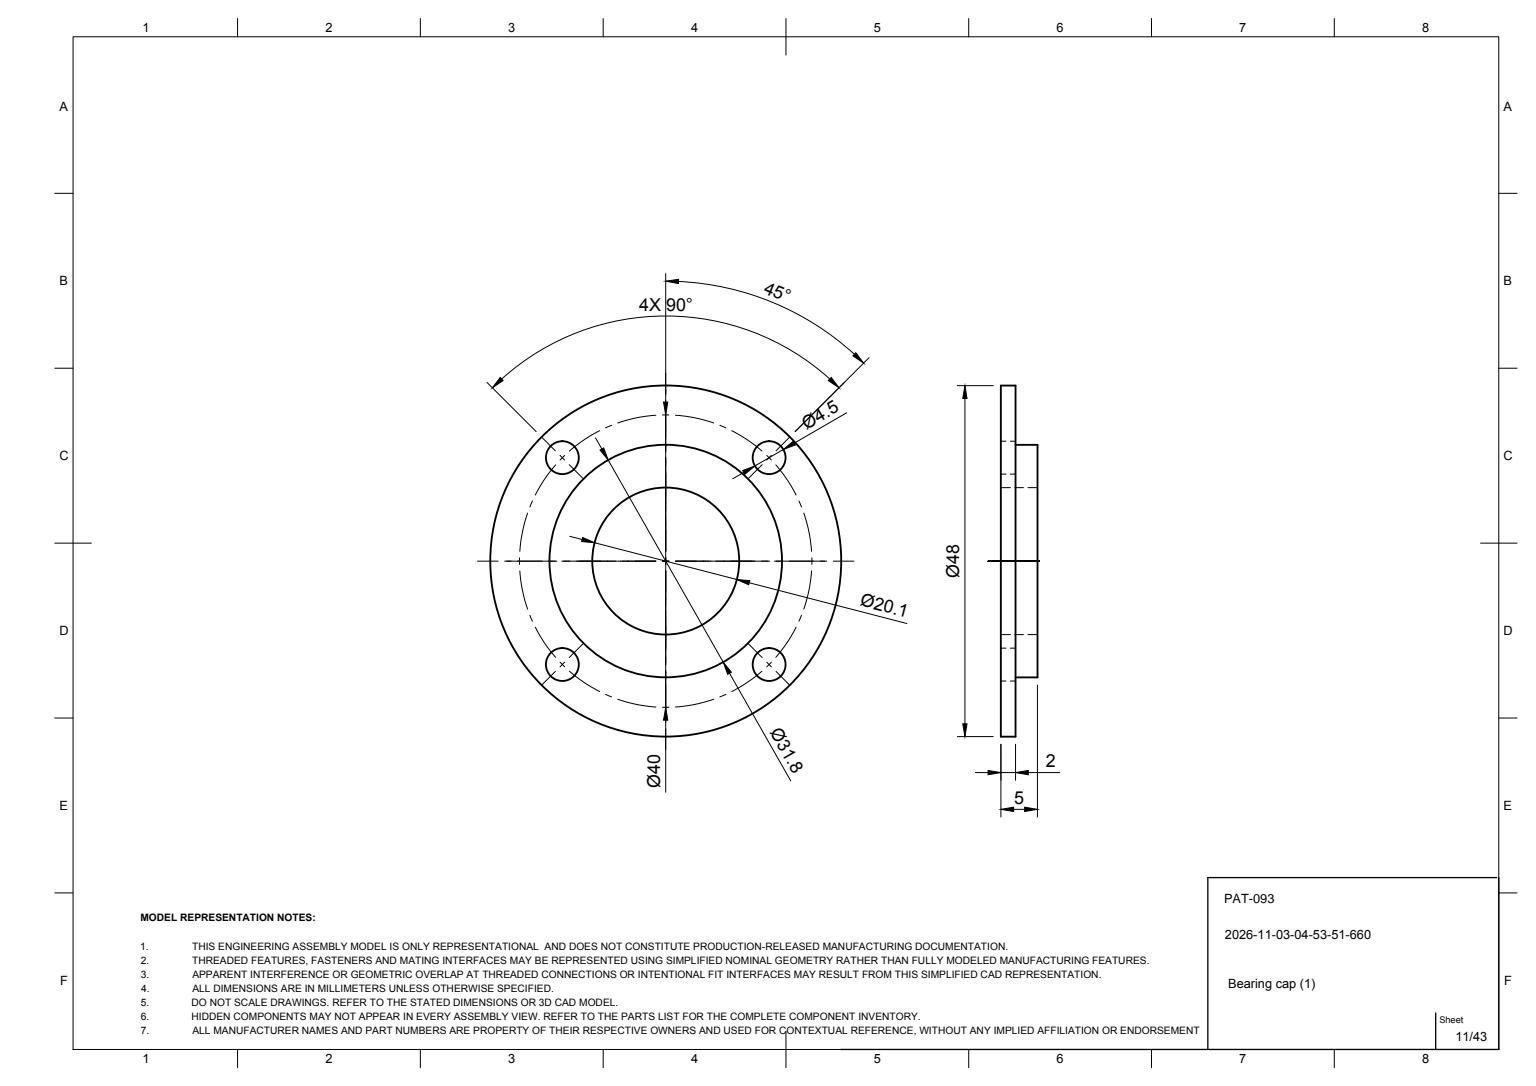
ISO-10303-21;
HEADER;
/* Generated by software containing ST-Developer
 * from STEP Tools, Inc. (www.steptools.com) 
 */

FILE_DESCRIPTION(
/* description */ ('Self-centering screw clamp'),
/* implementation_level */ '2;1');

FILE_NAME(
/* name */ 'Bearing cap (1).step',
/* time_stamp */ '2026-10-28T03:25:31-07:00',
/* author */ (''),
/* organization */ (''),
/* preprocessor_version */ 'ST-DEVELOPER v20.2',
/* originating_system */ 'Autodesk Translation Framework v15.17.0.0',
/* authorisation */ '');

FILE_SCHEMA (('AUTOMOTIVE_DESIGN { 1 0 10303 214 3 1 1 }'));
ENDSEC;

DATA;
#10=MECHANICAL_DESIGN_GEOMETRIC_PRESENTATION_REPRESENTATION('',(#633),#16799);
#551=SHAPE_REPRESENTATION_RELATIONSHIP('SRR','None',#17024,#592);
#592=ADVANCED_BREP_SHAPE_REPRESENTATION('',(#681),#16762);
#633=STYLED_ITEM('',(#17326),#681);
#681=MANIFOLD_SOLID_BREP('Body1',#9084);
#795=FACE_BOUND('',#1989,.T.);
#796=FACE_BOUND('',#1993,.T.);
#797=FACE_BOUND('',#1994,.T.);
#798=FACE_BOUND('',#1995,.T.);
#799=FACE_BOUND('',#1996,.T.);
#800=FACE_BOUND('',#1997,.T.);
#801=FACE_BOUND('',#1999,.T.);
#802=FACE_BOUND('',#2000,.T.);
#803=FACE_BOUND('',#2001,.T.);
#804=FACE_BOUND('',#2002,.T.);
#805=FACE_BOUND('',#2003,.T.);
#1085=PLANE('',#9853);
#1086=PLANE('',#9860);
#1087=PLANE('',#9861);
#1402=FACE_OUTER_BOUND('',#1983,.T.);
#1403=FACE_OUTER_BOUND('',#1984,.T.);
#1404=FACE_OUTER_BOUND('',#1985,.T.);
#1405=FACE_OUTER_BOUND('',#1986,.T.);
#1406=FACE_OUTER_BOUND('',#1987,.T.);
#1407=FACE_OUTER_BOUND('',#1988,.T.);
#1408=FACE_OUTER_BOUND('',#1990,.T.);
#1409=FACE_OUTER_BOUND('',#1991,.T.);
#1410=FACE_OUTER_BOUND('',#1992,.T.);
#1411=FACE_OUTER_BOUND('',#1998,.T.);
#1983=EDGE_LOOP('',(#6763,#6764,#6765,#6766));
#1984=EDGE_LOOP('',(#6767,#6768,#6769,#6770));
#1985=EDGE_LOOP('',(#6771,#6772,#6773,#6774));
#1986=EDGE_LOOP('',(#6775,#6776,#6777,#6778));
#1987=EDGE_LOOP('',(#6779,#6780,#6781,#6782));
#1988=EDGE_LOOP('',(#6783));
#1989=EDGE_LOOP('',(#6784));
#1990=EDGE_LOOP('',(#6785,#6786,#6787,#6788));
#1991=EDGE_LOOP('',(#6789,#6790,#6791,#6792));
#1992=EDGE_LOOP('',(#6793));
#1993=EDGE_LOOP('',(#6794));
#1994=EDGE_LOOP('',(#6795));
#1995=EDGE_LOOP('',(#6796));
#1996=EDGE_LOOP('',(#6797));
#1997=EDGE_LOOP('',(#6798));
#1998=EDGE_LOOP('',(#6799));
#1999=EDGE_LOOP('',(#6800));
#2000=EDGE_LOOP('',(#6801));
#2001=EDGE_LOOP('',(#6802));
#2002=EDGE_LOOP('',(#6803));
#2003=EDGE_LOOP('',(#6804));
#2771=LINE('',#14438,#3344);
#2772=LINE('',#14444,#3345);
#2773=LINE('',#14450,#3346);
#2774=LINE('',#14456,#3347);
#2775=LINE('',#14462,#3348);
#2776=LINE('',#14470,#3349);
#2777=LINE('',#14475,#3350);
#3344=VECTOR('',#11472,0.225);
#3345=VECTOR('',#11479,0.225);
#3346=VECTOR('',#11486,0.225);
#3347=VECTOR('',#11493,0.225);
#3348=VECTOR('',#11500,1.59);
#3349=VECTOR('',#11511,1.005);
#3350=VECTOR('',#11516,2.4);
#3843=CIRCLE('',#9839,0.225);
#3844=CIRCLE('',#9840,0.225);
#3845=CIRCLE('',#9842,0.225);
#3846=CIRCLE('',#9843,0.225);
#3847=CIRCLE('',#9845,0.225);
#3848=CIRCLE('',#9846,0.225);
#3849=CIRCLE('',#9848,0.225);
#3850=CIRCLE('',#9849,0.225);
#3851=CIRCLE('',#9851,1.59);
#3852=CIRCLE('',#9852,1.59);
#3853=CIRCLE('',#9854,1.005);
#3854=CIRCLE('',#9856,1.005);
#3855=CIRCLE('',#9858,2.4);
#3856=CIRCLE('',#9859,2.4);
#4441=VERTEX_POINT('',#14435);
#4442=VERTEX_POINT('',#14437);
#4443=VERTEX_POINT('',#14441);
#4444=VERTEX_POINT('',#14443);
#4445=VERTEX_POINT('',#14447);
#4446=VERTEX_POINT('',#14449);
#4447=VERTEX_POINT('',#14453);
#4448=VERTEX_POINT('',#14455);
#4449=VERTEX_POINT('',#14459);
#4450=VERTEX_POINT('',#14461);
#4451=VERTEX_POINT('',#14465);
#4452=VERTEX_POINT('',#14468);
#4453=VERTEX_POINT('',#14472);
#4454=VERTEX_POINT('',#14474);
#5306=EDGE_CURVE('',#4441,#4441,#3843,.T.);
#5307=EDGE_CURVE('',#4441,#4442,#2771,.T.);
#5308=EDGE_CURVE('',#4442,#4442,#3844,.T.);
#5309=EDGE_CURVE('',#4443,#4443,#3845,.T.);
#5310=EDGE_CURVE('',#4443,#4444,#2772,.T.);
#5311=EDGE_CURVE('',#4444,#4444,#3846,.T.);
#5312=EDGE_CURVE('',#4445,#4445,#3847,.T.);
#5313=EDGE_CURVE('',#4445,#4446,#2773,.T.);
#5314=EDGE_CURVE('',#4446,#4446,#3848,.T.);
#5315=EDGE_CURVE('',#4447,#4447,#3849,.T.);
#5316=EDGE_CURVE('',#4447,#4448,#2774,.T.);
#5317=EDGE_CURVE('',#4448,#4448,#3850,.T.);
#5318=EDGE_CURVE('',#4449,#4449,#3851,.T.);
#5319=EDGE_CURVE('',#4449,#4450,#2775,.T.);
#5320=EDGE_CURVE('',#4450,#4450,#3852,.T.);
#5321=EDGE_CURVE('',#4451,#4451,#3853,.T.);
#5322=EDGE_CURVE('',#4452,#4452,#3854,.T.);
#5323=EDGE_CURVE('',#4452,#4451,#2776,.T.);
#5324=EDGE_CURVE('',#4453,#4453,#3855,.T.);
#5325=EDGE_CURVE('',#4453,#4454,#2777,.T.);
#5326=EDGE_CURVE('',#4454,#4454,#3856,.T.);
#6763=ORIENTED_EDGE('',*,*,#5306,.F.);
#6764=ORIENTED_EDGE('',*,*,#5307,.T.);
#6765=ORIENTED_EDGE('',*,*,#5308,.F.);
#6766=ORIENTED_EDGE('',*,*,#5307,.F.);
#6767=ORIENTED_EDGE('',*,*,#5309,.F.);
#6768=ORIENTED_EDGE('',*,*,#5310,.T.);
#6769=ORIENTED_EDGE('',*,*,#5311,.F.);
#6770=ORIENTED_EDGE('',*,*,#5310,.F.);
#6771=ORIENTED_EDGE('',*,*,#5312,.F.);
#6772=ORIENTED_EDGE('',*,*,#5313,.T.);
#6773=ORIENTED_EDGE('',*,*,#5314,.F.);
#6774=ORIENTED_EDGE('',*,*,#5313,.F.);
#6775=ORIENTED_EDGE('',*,*,#5315,.F.);
#6776=ORIENTED_EDGE('',*,*,#5316,.T.);
#6777=ORIENTED_EDGE('',*,*,#5317,.F.);
#6778=ORIENTED_EDGE('',*,*,#5316,.F.);
#6779=ORIENTED_EDGE('',*,*,#5318,.F.);
#6780=ORIENTED_EDGE('',*,*,#5319,.T.);
#6781=ORIENTED_EDGE('',*,*,#5320,.T.);
#6782=ORIENTED_EDGE('',*,*,#5319,.F.);
#6783=ORIENTED_EDGE('',*,*,#5320,.F.);
#6784=ORIENTED_EDGE('',*,*,#5321,.F.);
#6785=ORIENTED_EDGE('',*,*,#5322,.F.);
#6786=ORIENTED_EDGE('',*,*,#5323,.T.);
#6787=ORIENTED_EDGE('',*,*,#5321,.T.);
#6788=ORIENTED_EDGE('',*,*,#5323,.F.);
#6789=ORIENTED_EDGE('',*,*,#5324,.F.);
#6790=ORIENTED_EDGE('',*,*,#5325,.T.);
#6791=ORIENTED_EDGE('',*,*,#5326,.T.);
#6792=ORIENTED_EDGE('',*,*,#5325,.F.);
#6793=ORIENTED_EDGE('',*,*,#5324,.T.);
#6794=ORIENTED_EDGE('',*,*,#5322,.T.);
#6795=ORIENTED_EDGE('',*,*,#5317,.T.);
#6796=ORIENTED_EDGE('',*,*,#5314,.T.);
#6797=ORIENTED_EDGE('',*,*,#5311,.T.);
#6798=ORIENTED_EDGE('',*,*,#5308,.T.);
#6799=ORIENTED_EDGE('',*,*,#5326,.F.);
#6800=ORIENTED_EDGE('',*,*,#5318,.T.);
#6801=ORIENTED_EDGE('',*,*,#5315,.T.);
#6802=ORIENTED_EDGE('',*,*,#5312,.T.);
#6803=ORIENTED_EDGE('',*,*,#5309,.T.);
#6804=ORIENTED_EDGE('',*,*,#5306,.T.);
#8415=CYLINDRICAL_SURFACE('',#9838,0.225);
#8416=CYLINDRICAL_SURFACE('',#9841,0.225);
#8417=CYLINDRICAL_SURFACE('',#9844,0.225);
#8418=CYLINDRICAL_SURFACE('',#9847,0.225);
#8419=CYLINDRICAL_SURFACE('',#9850,1.59);
#8420=CYLINDRICAL_SURFACE('',#9855,1.005);
#8421=CYLINDRICAL_SURFACE('',#9857,2.4);
#8700=ADVANCED_FACE('',(#1402),#8415,.F.);
#8701=ADVANCED_FACE('',(#1403),#8416,.F.);
#8702=ADVANCED_FACE('',(#1404),#8417,.F.);
#8703=ADVANCED_FACE('',(#1405),#8418,.F.);
#8704=ADVANCED_FACE('',(#1406),#8419,.T.);
#8705=ADVANCED_FACE('',(#1407,#795),#1085,.F.);
#8706=ADVANCED_FACE('',(#1408),#8420,.F.);
#8707=ADVANCED_FACE('',(#1409),#8421,.T.);
#8708=ADVANCED_FACE('',(#1410,#796,#797,#798,#799,#800),#1086,.T.);
#8709=ADVANCED_FACE('',(#1411,#801,#802,#803,#804,#805),#1087,.F.);
#9084=CLOSED_SHELL('',(#8700,#8701,#8702,#8703,#8704,#8705,#8706,#8707,
#8708,#8709));
#9837=AXIS2_PLACEMENT_3D('',#14433,#11466,#11467);
#9838=AXIS2_PLACEMENT_3D('',#14434,#11468,#11469);
#9839=AXIS2_PLACEMENT_3D('',#14436,#11470,#11471);
#9840=AXIS2_PLACEMENT_3D('',#14439,#11473,#11474);
#9841=AXIS2_PLACEMENT_3D('',#14440,#11475,#11476);
#9842=AXIS2_PLACEMENT_3D('',#14442,#11477,#11478);
#9843=AXIS2_PLACEMENT_3D('',#14445,#11480,#11481);
#9844=AXIS2_PLACEMENT_3D('',#14446,#11482,#11483);
#9845=AXIS2_PLACEMENT_3D('',#14448,#11484,#11485);
#9846=AXIS2_PLACEMENT_3D('',#14451,#11487,#11488);
#9847=AXIS2_PLACEMENT_3D('',#14452,#11489,#11490);
#9848=AXIS2_PLACEMENT_3D('',#14454,#11491,#11492);
#9849=AXIS2_PLACEMENT_3D('',#14457,#11494,#11495);
#9850=AXIS2_PLACEMENT_3D('',#14458,#11496,#11497);
#9851=AXIS2_PLACEMENT_3D('',#14460,#11498,#11499);
#9852=AXIS2_PLACEMENT_3D('',#14463,#11501,#11502);
#9853=AXIS2_PLACEMENT_3D('',#14464,#11503,#11504);
#9854=AXIS2_PLACEMENT_3D('',#14466,#11505,#11506);
#9855=AXIS2_PLACEMENT_3D('',#14467,#11507,#11508);
#9856=AXIS2_PLACEMENT_3D('',#14469,#11509,#11510);
#9857=AXIS2_PLACEMENT_3D('',#14471,#11512,#11513);
#9858=AXIS2_PLACEMENT_3D('',#14473,#11514,#11515);
#9859=AXIS2_PLACEMENT_3D('',#14476,#11517,#11518);
#9860=AXIS2_PLACEMENT_3D('',#14477,#11519,#11520);
#9861=AXIS2_PLACEMENT_3D('',#14478,#11521,#11522);
#11466=DIRECTION('axis',(0.,0.,1.));
#11467=DIRECTION('refdir',(1.,0.,0.));
#11468=DIRECTION('center_axis',(1.,0.,0.));
#11469=DIRECTION('ref_axis',(0.,0.,-1.));
#11470=DIRECTION('center_axis',(1.,0.,0.));
#11471=DIRECTION('ref_axis',(0.,0.,-1.));
#11472=DIRECTION('',(1.,0.,0.));
#11473=DIRECTION('center_axis',(-1.,0.,0.));
#11474=DIRECTION('ref_axis',(0.,0.,-1.));
#11475=DIRECTION('center_axis',(1.,0.,0.));
#11476=DIRECTION('ref_axis',(0.,0.,-1.));
#11477=DIRECTION('center_axis',(1.,0.,0.));
#11478=DIRECTION('ref_axis',(0.,0.,-1.));
#11479=DIRECTION('',(1.,0.,0.));
#11480=DIRECTION('center_axis',(-1.,0.,0.));
#11481=DIRECTION('ref_axis',(0.,0.,-1.));
#11482=DIRECTION('center_axis',(1.,0.,0.));
#11483=DIRECTION('ref_axis',(0.,0.,-1.));
#11484=DIRECTION('center_axis',(1.,0.,0.));
#11485=DIRECTION('ref_axis',(0.,0.,-1.));
#11486=DIRECTION('',(1.,0.,0.));
#11487=DIRECTION('center_axis',(-1.,0.,0.));
#11488=DIRECTION('ref_axis',(0.,0.,-1.));
#11489=DIRECTION('center_axis',(1.,0.,0.));
#11490=DIRECTION('ref_axis',(0.,0.,-1.));
#11491=DIRECTION('center_axis',(1.,0.,0.));
#11492=DIRECTION('ref_axis',(0.,0.,-1.));
#11493=DIRECTION('',(1.,0.,0.));
#11494=DIRECTION('center_axis',(-1.,0.,0.));
#11495=DIRECTION('ref_axis',(0.,0.,-1.));
#11496=DIRECTION('center_axis',(1.,0.,0.));
#11497=DIRECTION('ref_axis',(0.,0.,-1.));
#11498=DIRECTION('center_axis',(1.,0.,0.));
#11499=DIRECTION('ref_axis',(0.,0.,-1.));
#11500=DIRECTION('',(-1.,0.,0.));
#11501=DIRECTION('center_axis',(1.,0.,0.));
#11502=DIRECTION('ref_axis',(0.,0.,-1.));
#11503=DIRECTION('center_axis',(1.,0.,0.));
#11504=DIRECTION('ref_axis',(0.,0.,-1.));
#11505=DIRECTION('center_axis',(-1.,0.,0.));
#11506=DIRECTION('ref_axis',(0.,0.,-1.));
#11507=DIRECTION('center_axis',(1.,0.,0.));
#11508=DIRECTION('ref_axis',(0.,0.,-1.));
#11509=DIRECTION('center_axis',(-1.,0.,0.));
#11510=DIRECTION('ref_axis',(0.,0.,-1.));
#11511=DIRECTION('',(-1.,0.,0.));
#11512=DIRECTION('center_axis',(1.,0.,0.));
#11513=DIRECTION('ref_axis',(0.,0.,-1.));
#11514=DIRECTION('center_axis',(1.,0.,0.));
#11515=DIRECTION('ref_axis',(0.,0.,-1.));
#11516=DIRECTION('',(-1.,0.,0.));
#11517=DIRECTION('center_axis',(1.,0.,0.));
#11518=DIRECTION('ref_axis',(0.,0.,-1.));
#11519=DIRECTION('center_axis',(1.,0.,0.));
#11520=DIRECTION('ref_axis',(0.,0.,-1.));
#11521=DIRECTION('center_axis',(1.,0.,0.));
#11522=DIRECTION('ref_axis',(0.,0.,-1.));
#14433=CARTESIAN_POINT('',(0.,0.,0.));
#14434=CARTESIAN_POINT('Origin',(-10.8,-1.4142135623731,2.58578643762691));
#14435=CARTESIAN_POINT('',(-10.7,-1.4142135623731,2.81078643762691));
#14436=CARTESIAN_POINT('Origin',(-10.7,-1.4142135623731,2.58578643762691));
#14437=CARTESIAN_POINT('',(-10.5,-1.4142135623731,2.81078643762691));
#14438=CARTESIAN_POINT('',(-10.8,-1.4142135623731,2.81078643762691));
#14439=CARTESIAN_POINT('Origin',(-10.5,-1.4142135623731,2.58578643762691));
#14440=CARTESIAN_POINT('Origin',(-10.8,-1.41421356237309,5.41421356237309));
#14441=CARTESIAN_POINT('',(-10.7,-1.41421356237309,5.63921356237309));
#14442=CARTESIAN_POINT('Origin',(-10.7,-1.41421356237309,5.41421356237309));
#14443=CARTESIAN_POINT('',(-10.5,-1.41421356237309,5.63921356237309));
#14444=CARTESIAN_POINT('',(-10.8,-1.41421356237309,5.63921356237309));
#14445=CARTESIAN_POINT('Origin',(-10.5,-1.41421356237309,5.41421356237309));
#14446=CARTESIAN_POINT('Origin',(-10.8,1.4142135623731,5.41421356237309));
#14447=CARTESIAN_POINT('',(-10.7,1.4142135623731,5.63921356237309));
#14448=CARTESIAN_POINT('Origin',(-10.7,1.4142135623731,5.41421356237309));
#14449=CARTESIAN_POINT('',(-10.5,1.4142135623731,5.63921356237309));
#14450=CARTESIAN_POINT('',(-10.8,1.4142135623731,5.63921356237309));
#14451=CARTESIAN_POINT('Origin',(-10.5,1.4142135623731,5.41421356237309));
#14452=CARTESIAN_POINT('Origin',(-10.8,1.41421356237309,2.5857864376269));
#14453=CARTESIAN_POINT('',(-10.7,1.41421356237309,2.8107864376269));
#14454=CARTESIAN_POINT('Origin',(-10.7,1.41421356237309,2.5857864376269));
#14455=CARTESIAN_POINT('',(-10.5,1.41421356237309,2.8107864376269));
#14456=CARTESIAN_POINT('',(-10.8,1.41421356237309,2.8107864376269));
#14457=CARTESIAN_POINT('Origin',(-10.5,1.41421356237309,2.5857864376269));
#14458=CARTESIAN_POINT('Origin',(-11.,0.,4.));
#14459=CARTESIAN_POINT('',(-10.7,-1.94718841064429E-16,5.59));
#14460=CARTESIAN_POINT('Origin',(-10.7,0.,4.));
#14461=CARTESIAN_POINT('',(-11.,-1.94718841064429E-16,5.59));
#14462=CARTESIAN_POINT('',(-11.,-1.94718841064429E-16,5.59));
#14463=CARTESIAN_POINT('Origin',(-11.,0.,4.));
#14464=CARTESIAN_POINT('Origin',(-11.,0.,4.));
#14465=CARTESIAN_POINT('',(-11.,-1.23077003314309E-16,5.005));
#14466=CARTESIAN_POINT('Origin',(-11.,0.,4.));
#14467=CARTESIAN_POINT('Origin',(-10.7,0.,4.));
#14468=CARTESIAN_POINT('',(-10.5,-1.23077003314309E-16,5.005));
#14469=CARTESIAN_POINT('Origin',(-10.5,0.,4.));
#14470=CARTESIAN_POINT('',(-10.7,-1.23077003314309E-16,5.005));
#14471=CARTESIAN_POINT('Origin',(-10.7,0.,4.));
#14472=CARTESIAN_POINT('',(-10.5,-2.93915231795365E-16,6.4));
#14473=CARTESIAN_POINT('Origin',(-10.5,0.,4.));
#14474=CARTESIAN_POINT('',(-10.7,-2.93915231795365E-16,6.4));
#14475=CARTESIAN_POINT('',(-10.7,-2.93915231795365E-16,6.4));
#14476=CARTESIAN_POINT('Origin',(-10.7,0.,4.));
#14477=CARTESIAN_POINT('Origin',(-10.5,0.,4.));
#14478=CARTESIAN_POINT('Origin',(-10.7,0.,4.));
#16713=UNCERTAINTY_MEASURE_WITH_UNIT(LENGTH_MEASURE(0.001),#16800,
'DISTANCE_ACCURACY_VALUE',
'Maximum model space distance between geometric entities at asserted c
onnectivities');
#16750=UNCERTAINTY_MEASURE_WITH_UNIT(LENGTH_MEASURE(0.001),#16800,
'DISTANCE_ACCURACY_VALUE',
'Maximum model space distance between geometric entities at asserted c
onnectivities');
#16762=(
GEOMETRIC_REPRESENTATION_CONTEXT(3)
GLOBAL_UNCERTAINTY_ASSIGNED_CONTEXT((#16713))
GLOBAL_UNIT_ASSIGNED_CONTEXT((#16800,#16802,#16803))
REPRESENTATION_CONTEXT('','3D')
);
#16799=(
GEOMETRIC_REPRESENTATION_CONTEXT(3)
GLOBAL_UNCERTAINTY_ASSIGNED_CONTEXT((#16750))
GLOBAL_UNIT_ASSIGNED_CONTEXT((#16800,#16802,#16803))
REPRESENTATION_CONTEXT('','3D')
);
#16800=(
LENGTH_UNIT()
NAMED_UNIT(*)
SI_UNIT(.CENTI.,.METRE.)
);
#16802=(
NAMED_UNIT(*)
PLANE_ANGLE_UNIT()
SI_UNIT($,.RADIAN.)
);
#16803=(
NAMED_UNIT(*)
SI_UNIT($,.STERADIAN.)
SOLID_ANGLE_UNIT()
);
#16815=SHAPE_DEFINITION_REPRESENTATION(#16863,#17024);
#16863=PRODUCT_DEFINITION_SHAPE('',$,#17073);
#17024=SHAPE_REPRESENTATION('',(#9837),#16762);
#17061=PRODUCT_DEFINITION_CONTEXT('part definition',#17207,'design');
#17073=PRODUCT_DEFINITION('Bearing cap (1)','Bearing cap (1)',#17121,#17061);
#17121=PRODUCT_DEFINITION_FORMATION('',$,#17220);
#17207=APPLICATION_CONTEXT(
'Core Data for Automotive Mechanical Design Process');
#17208=PRODUCT_CONTEXT('part definition',#17207,'mechanical');
#17220=PRODUCT('Bearing cap (1)','Bearing cap (1)','Bearing cap (1)',(#17208));
#17320=COLOUR_RGB('Grey',0.48,0.52,0.57);
#17321=FILL_AREA_STYLE_COLOUR('',#17320);
#17322=FILL_AREA_STYLE('',(#17321));
#17323=SURFACE_STYLE_FILL_AREA(#17322);
#17324=SURFACE_SIDE_STYLE('',(#17323));
#17325=SURFACE_STYLE_USAGE(.BOTH.,#17324);
#17326=PRESENTATION_STYLE_ASSIGNMENT((#17325));
ENDSEC;
END-ISO-10303-21;
